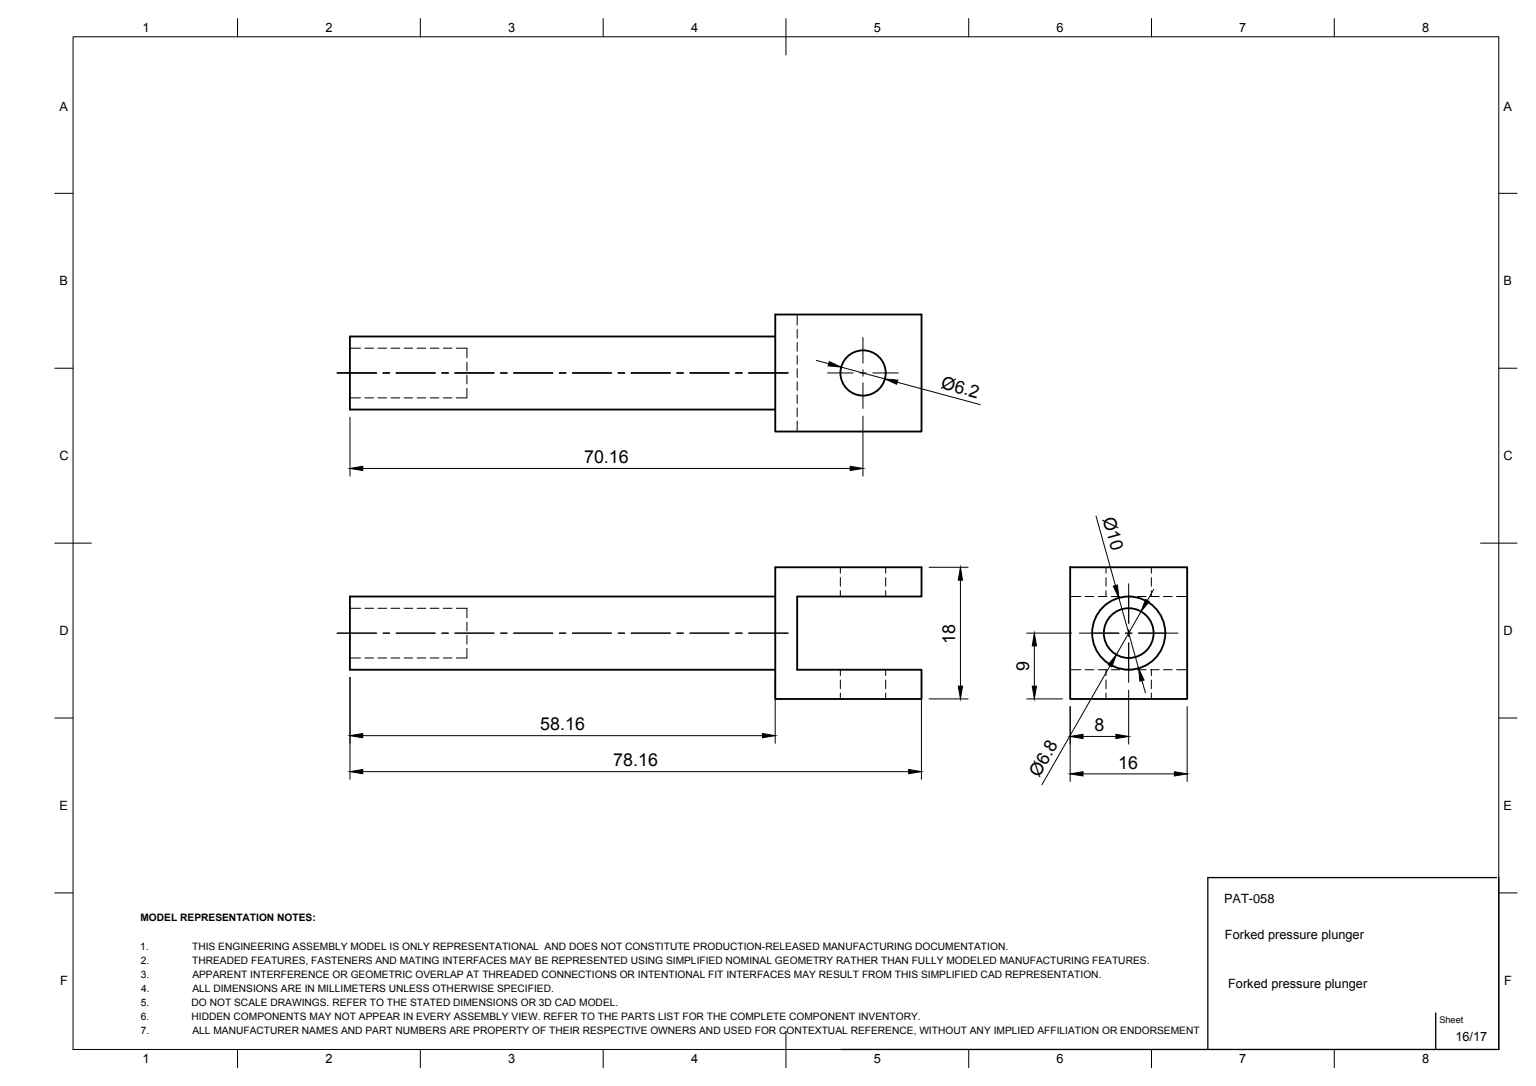
ISO-10303-21;
HEADER;
/* Generated by software containing ST-Developer
 * from STEP Tools, Inc. (www.steptools.com) 
 */

FILE_DESCRIPTION(
/* description */ ('Horizontal push-pull toggle clamp'),
/* implementation_level */ '2;1');

FILE_NAME(
/* name */ 'Forked pressure plunger.step',
/* time_stamp */ '2026-10-27T21:21:09-07:00',
/* author */ (''),
/* organization */ (''),
/* preprocessor_version */ 'ST-DEVELOPER v20.2',
/* originating_system */ 'Autodesk Translation Framework v15.17.0.0',
/* authorisation */ '');

FILE_SCHEMA (('AUTOMOTIVE_DESIGN { 1 0 10303 214 3 1 1 }'));
ENDSEC;

DATA;
#10=MECHANICAL_DESIGN_GEOMETRIC_PRESENTATION_REPRESENTATION('',(#190),#4791);
#164=SHAPE_REPRESENTATION_RELATIONSHIP('SRR','None',#4870,#177);
#177=ADVANCED_BREP_SHAPE_REPRESENTATION('',(#202),#4783);
#190=STYLED_ITEM('',(#5009),#202);
#202=MANIFOLD_SOLID_BREP('Body1',#2635);
#240=FACE_BOUND('',#637,.T.);
#241=FACE_BOUND('',#640,.T.);
#242=FACE_BOUND('',#643,.T.);
#243=FACE_BOUND('',#646,.T.);
#244=FACE_BOUND('',#649,.T.);
#245=FACE_BOUND('',#652,.T.);
#321=PLANE('',#2939);
#322=PLANE('',#2946);
#323=PLANE('',#2947);
#324=PLANE('',#2948);
#325=PLANE('',#2949);
#326=PLANE('',#2950);
#327=PLANE('',#2951);
#328=PLANE('',#2953);
#329=PLANE('',#2954);
#330=PLANE('',#2955);
#331=PLANE('',#2956);
#332=PLANE('',#2959);
#450=FACE_OUTER_BOUND('',#631,.T.);
#451=FACE_OUTER_BOUND('',#632,.T.);
#452=FACE_OUTER_BOUND('',#633,.T.);
#453=FACE_OUTER_BOUND('',#634,.T.);
#454=FACE_OUTER_BOUND('',#635,.T.);
#455=FACE_OUTER_BOUND('',#636,.T.);
#456=FACE_OUTER_BOUND('',#638,.T.);
#457=FACE_OUTER_BOUND('',#639,.T.);
#458=FACE_OUTER_BOUND('',#641,.T.);
#459=FACE_OUTER_BOUND('',#642,.T.);
#460=FACE_OUTER_BOUND('',#644,.T.);
#461=FACE_OUTER_BOUND('',#645,.T.);
#462=FACE_OUTER_BOUND('',#647,.T.);
#463=FACE_OUTER_BOUND('',#648,.T.);
#464=FACE_OUTER_BOUND('',#650,.T.);
#465=FACE_OUTER_BOUND('',#651,.T.);
#631=EDGE_LOOP('',(#2185,#2186,#2187,#2188));
#632=EDGE_LOOP('',(#2189));
#633=EDGE_LOOP('',(#2190,#2191,#2192,#2193));
#634=EDGE_LOOP('',(#2194,#2195,#2196,#2197));
#635=EDGE_LOOP('',(#2198,#2199,#2200,#2201));
#636=EDGE_LOOP('',(#2202,#2203,#2204,#2205));
#637=EDGE_LOOP('',(#2206));
#638=EDGE_LOOP('',(#2207,#2208,#2209,#2210,#2211,#2212,#2213,#2214));
#639=EDGE_LOOP('',(#2215,#2216,#2217,#2218));
#640=EDGE_LOOP('',(#2219));
#641=EDGE_LOOP('',(#2220,#2221,#2222,#2223));
#642=EDGE_LOOP('',(#2224,#2225,#2226,#2227));
#643=EDGE_LOOP('',(#2228));
#644=EDGE_LOOP('',(#2229,#2230,#2231,#2232,#2233,#2234,#2235,#2236));
#645=EDGE_LOOP('',(#2237,#2238,#2239,#2240));
#646=EDGE_LOOP('',(#2241));
#647=EDGE_LOOP('',(#2242,#2243,#2244,#2245));
#648=EDGE_LOOP('',(#2246,#2247,#2248,#2249));
#649=EDGE_LOOP('',(#2250));
#650=EDGE_LOOP('',(#2251,#2252,#2253,#2254));
#651=EDGE_LOOP('',(#2255));
#652=EDGE_LOOP('',(#2256));
#759=CIRCLE('',#2937,0.34);
#760=CIRCLE('',#2938,0.34);
#761=CIRCLE('',#2941,0.31);
#762=CIRCLE('',#2942,0.31);
#763=CIRCLE('',#2944,0.31);
#764=CIRCLE('',#2945,0.31);
#765=CIRCLE('',#2952,0.5);
#766=CIRCLE('',#2958,0.5);
#948=LINE('',#4294,#1168);
#949=LINE('',#4301,#1169);
#950=LINE('',#4307,#1170);
#951=LINE('',#4312,#1171);
#952=LINE('',#4314,#1172);
#953=LINE('',#4316,#1173);
#954=LINE('',#4317,#1174);
#955=LINE('',#4321,#1175);
#956=LINE('',#4323,#1176);
#957=LINE('',#4325,#1177);
#958=LINE('',#4326,#1178);
#959=LINE('',#4329,#1179);
#960=LINE('',#4330,#1180);
#961=LINE('',#4332,#1181);
#962=LINE('',#4334,#1182);
#963=LINE('',#4336,#1183);
#964=LINE('',#4337,#1184);
#965=LINE('',#4341,#1185);
#966=LINE('',#4342,#1186);
#967=LINE('',#4343,#1187);
#968=LINE('',#4346,#1188);
#969=LINE('',#4347,#1189);
#970=LINE('',#4349,#1190);
#971=LINE('',#4353,#1191);
#972=LINE('',#4355,#1192);
#973=LINE('',#4356,#1193);
#974=LINE('',#4359,#1194);
#975=LINE('',#4364,#1195);
#1168=VECTOR('',#3524,0.34);
#1169=VECTOR('',#3533,0.31);
#1170=VECTOR('',#3540,0.31);
#1171=VECTOR('',#3545,1.);
#1172=VECTOR('',#3546,1.);
#1173=VECTOR('',#3547,1.);
#1174=VECTOR('',#3548,1.);
#1175=VECTOR('',#3551,1.);
#1176=VECTOR('',#3552,1.);
#1177=VECTOR('',#3553,1.);
#1178=VECTOR('',#3554,1.);
#1179=VECTOR('',#3557,1.);
#1180=VECTOR('',#3558,1.);
#1181=VECTOR('',#3559,1.);
#1182=VECTOR('',#3560,1.);
#1183=VECTOR('',#3561,1.);
#1184=VECTOR('',#3562,1.);
#1185=VECTOR('',#3565,1.);
#1186=VECTOR('',#3566,1.);
#1187=VECTOR('',#3567,1.);
#1188=VECTOR('',#3570,1.);
#1189=VECTOR('',#3571,1.);
#1190=VECTOR('',#3574,1.);
#1191=VECTOR('',#3579,1.);
#1192=VECTOR('',#3580,1.);
#1193=VECTOR('',#3581,1.);
#1194=VECTOR('',#3586,1.);
#1195=VECTOR('',#3593,0.5);
#1369=VERTEX_POINT('',#4291);
#1370=VERTEX_POINT('',#4293);
#1371=VERTEX_POINT('',#4298);
#1372=VERTEX_POINT('',#4300);
#1373=VERTEX_POINT('',#4304);
#1374=VERTEX_POINT('',#4306);
#1375=VERTEX_POINT('',#4310);
#1376=VERTEX_POINT('',#4311);
#1377=VERTEX_POINT('',#4313);
#1378=VERTEX_POINT('',#4315);
#1379=VERTEX_POINT('',#4319);
#1380=VERTEX_POINT('',#4320);
#1381=VERTEX_POINT('',#4322);
#1382=VERTEX_POINT('',#4324);
#1383=VERTEX_POINT('',#4328);
#1384=VERTEX_POINT('',#4331);
#1385=VERTEX_POINT('',#4333);
#1386=VERTEX_POINT('',#4335);
#1387=VERTEX_POINT('',#4339);
#1388=VERTEX_POINT('',#4340);
#1389=VERTEX_POINT('',#4345);
#1390=VERTEX_POINT('',#4350);
#1391=VERTEX_POINT('',#4354);
#1392=VERTEX_POINT('',#4362);
#1654=EDGE_CURVE('',#1369,#1369,#759,.T.);
#1655=EDGE_CURVE('',#1369,#1370,#948,.T.);
#1656=EDGE_CURVE('',#1370,#1370,#760,.T.);
#1657=EDGE_CURVE('',#1371,#1371,#761,.T.);
#1658=EDGE_CURVE('',#1371,#1372,#949,.T.);
#1659=EDGE_CURVE('',#1372,#1372,#762,.T.);
#1660=EDGE_CURVE('',#1373,#1373,#763,.T.);
#1661=EDGE_CURVE('',#1373,#1374,#950,.T.);
#1662=EDGE_CURVE('',#1374,#1374,#764,.T.);
#1663=EDGE_CURVE('',#1375,#1376,#951,.T.);
#1664=EDGE_CURVE('',#1377,#1375,#952,.T.);
#1665=EDGE_CURVE('',#1378,#1377,#953,.T.);
#1666=EDGE_CURVE('',#1378,#1376,#954,.T.);
#1667=EDGE_CURVE('',#1379,#1380,#955,.T.);
#1668=EDGE_CURVE('',#1380,#1381,#956,.T.);
#1669=EDGE_CURVE('',#1381,#1382,#957,.T.);
#1670=EDGE_CURVE('',#1382,#1379,#958,.T.);
#1671=EDGE_CURVE('',#1383,#1375,#959,.T.);
#1672=EDGE_CURVE('',#1383,#1380,#960,.T.);
#1673=EDGE_CURVE('',#1384,#1379,#961,.T.);
#1674=EDGE_CURVE('',#1385,#1384,#962,.T.);
#1675=EDGE_CURVE('',#1385,#1386,#963,.T.);
#1676=EDGE_CURVE('',#1377,#1386,#964,.T.);
#1677=EDGE_CURVE('',#1387,#1388,#965,.T.);
#1678=EDGE_CURVE('',#1388,#1385,#966,.T.);
#1679=EDGE_CURVE('',#1384,#1387,#967,.T.);
#1680=EDGE_CURVE('',#1389,#1383,#968,.T.);
#1681=EDGE_CURVE('',#1389,#1381,#969,.T.);
#1682=EDGE_CURVE('',#1387,#1382,#970,.T.);
#1683=EDGE_CURVE('',#1390,#1390,#765,.T.);
#1684=EDGE_CURVE('',#1376,#1389,#971,.T.);
#1685=EDGE_CURVE('',#1391,#1378,#972,.T.);
#1686=EDGE_CURVE('',#1388,#1391,#973,.T.);
#1687=EDGE_CURVE('',#1386,#1391,#974,.T.);
#1688=EDGE_CURVE('',#1392,#1392,#766,.T.);
#1689=EDGE_CURVE('',#1392,#1390,#975,.T.);
#2185=ORIENTED_EDGE('',*,*,#1654,.F.);
#2186=ORIENTED_EDGE('',*,*,#1655,.T.);
#2187=ORIENTED_EDGE('',*,*,#1656,.F.);
#2188=ORIENTED_EDGE('',*,*,#1655,.F.);
#2189=ORIENTED_EDGE('',*,*,#1654,.T.);
#2190=ORIENTED_EDGE('',*,*,#1657,.F.);
#2191=ORIENTED_EDGE('',*,*,#1658,.T.);
#2192=ORIENTED_EDGE('',*,*,#1659,.F.);
#2193=ORIENTED_EDGE('',*,*,#1658,.F.);
#2194=ORIENTED_EDGE('',*,*,#1660,.F.);
#2195=ORIENTED_EDGE('',*,*,#1661,.T.);
#2196=ORIENTED_EDGE('',*,*,#1662,.F.);
#2197=ORIENTED_EDGE('',*,*,#1661,.F.);
#2198=ORIENTED_EDGE('',*,*,#1663,.F.);
#2199=ORIENTED_EDGE('',*,*,#1664,.F.);
#2200=ORIENTED_EDGE('',*,*,#1665,.F.);
#2201=ORIENTED_EDGE('',*,*,#1666,.T.);
#2202=ORIENTED_EDGE('',*,*,#1667,.T.);
#2203=ORIENTED_EDGE('',*,*,#1668,.T.);
#2204=ORIENTED_EDGE('',*,*,#1669,.T.);
#2205=ORIENTED_EDGE('',*,*,#1670,.T.);
#2206=ORIENTED_EDGE('',*,*,#1662,.T.);
#2207=ORIENTED_EDGE('',*,*,#1671,.F.);
#2208=ORIENTED_EDGE('',*,*,#1672,.T.);
#2209=ORIENTED_EDGE('',*,*,#1667,.F.);
#2210=ORIENTED_EDGE('',*,*,#1673,.F.);
#2211=ORIENTED_EDGE('',*,*,#1674,.F.);
#2212=ORIENTED_EDGE('',*,*,#1675,.T.);
#2213=ORIENTED_EDGE('',*,*,#1676,.F.);
#2214=ORIENTED_EDGE('',*,*,#1664,.T.);
#2215=ORIENTED_EDGE('',*,*,#1677,.T.);
#2216=ORIENTED_EDGE('',*,*,#1678,.T.);
#2217=ORIENTED_EDGE('',*,*,#1674,.T.);
#2218=ORIENTED_EDGE('',*,*,#1679,.T.);
#2219=ORIENTED_EDGE('',*,*,#1657,.T.);
#2220=ORIENTED_EDGE('',*,*,#1680,.F.);
#2221=ORIENTED_EDGE('',*,*,#1681,.T.);
#2222=ORIENTED_EDGE('',*,*,#1668,.F.);
#2223=ORIENTED_EDGE('',*,*,#1672,.F.);
#2224=ORIENTED_EDGE('',*,*,#1673,.T.);
#2225=ORIENTED_EDGE('',*,*,#1670,.F.);
#2226=ORIENTED_EDGE('',*,*,#1682,.F.);
#2227=ORIENTED_EDGE('',*,*,#1679,.F.);
#2228=ORIENTED_EDGE('',*,*,#1683,.F.);
#2229=ORIENTED_EDGE('',*,*,#1669,.F.);
#2230=ORIENTED_EDGE('',*,*,#1681,.F.);
#2231=ORIENTED_EDGE('',*,*,#1684,.F.);
#2232=ORIENTED_EDGE('',*,*,#1666,.F.);
#2233=ORIENTED_EDGE('',*,*,#1685,.F.);
#2234=ORIENTED_EDGE('',*,*,#1686,.F.);
#2235=ORIENTED_EDGE('',*,*,#1677,.F.);
#2236=ORIENTED_EDGE('',*,*,#1682,.T.);
#2237=ORIENTED_EDGE('',*,*,#1663,.T.);
#2238=ORIENTED_EDGE('',*,*,#1684,.T.);
#2239=ORIENTED_EDGE('',*,*,#1680,.T.);
#2240=ORIENTED_EDGE('',*,*,#1671,.T.);
#2241=ORIENTED_EDGE('',*,*,#1660,.T.);
#2242=ORIENTED_EDGE('',*,*,#1678,.F.);
#2243=ORIENTED_EDGE('',*,*,#1686,.T.);
#2244=ORIENTED_EDGE('',*,*,#1687,.F.);
#2245=ORIENTED_EDGE('',*,*,#1675,.F.);
#2246=ORIENTED_EDGE('',*,*,#1665,.T.);
#2247=ORIENTED_EDGE('',*,*,#1676,.T.);
#2248=ORIENTED_EDGE('',*,*,#1687,.T.);
#2249=ORIENTED_EDGE('',*,*,#1685,.T.);
#2250=ORIENTED_EDGE('',*,*,#1659,.T.);
#2251=ORIENTED_EDGE('',*,*,#1688,.F.);
#2252=ORIENTED_EDGE('',*,*,#1689,.T.);
#2253=ORIENTED_EDGE('',*,*,#1683,.T.);
#2254=ORIENTED_EDGE('',*,*,#1689,.F.);
#2255=ORIENTED_EDGE('',*,*,#1688,.T.);
#2256=ORIENTED_EDGE('',*,*,#1656,.T.);
#2463=CYLINDRICAL_SURFACE('',#2936,0.34);
#2464=CYLINDRICAL_SURFACE('',#2940,0.31);
#2465=CYLINDRICAL_SURFACE('',#2943,0.31);
#2466=CYLINDRICAL_SURFACE('',#2957,0.5);
#2566=ADVANCED_FACE('',(#450),#2463,.F.);
#2567=ADVANCED_FACE('',(#451),#321,.T.);
#2568=ADVANCED_FACE('',(#452),#2464,.F.);
#2569=ADVANCED_FACE('',(#453),#2465,.F.);
#2570=ADVANCED_FACE('',(#454),#322,.T.);
#2571=ADVANCED_FACE('',(#455,#240),#323,.T.);
#2572=ADVANCED_FACE('',(#456),#324,.T.);
#2573=ADVANCED_FACE('',(#457,#241),#325,.F.);
#2574=ADVANCED_FACE('',(#458),#326,.T.);
#2575=ADVANCED_FACE('',(#459,#242),#327,.T.);
#2576=ADVANCED_FACE('',(#460),#328,.T.);
#2577=ADVANCED_FACE('',(#461,#243),#329,.F.);
#2578=ADVANCED_FACE('',(#462),#330,.T.);
#2579=ADVANCED_FACE('',(#463,#244),#331,.T.);
#2580=ADVANCED_FACE('',(#464),#2466,.T.);
#2581=ADVANCED_FACE('',(#465,#245),#332,.T.);
#2635=CLOSED_SHELL('',(#2566,#2567,#2568,#2569,#2570,#2571,#2572,#2573,
#2574,#2575,#2576,#2577,#2578,#2579,#2580,#2581));
#2935=AXIS2_PLACEMENT_3D('',#4289,#3518,#3519);
#2936=AXIS2_PLACEMENT_3D('',#4290,#3520,#3521);
#2937=AXIS2_PLACEMENT_3D('',#4292,#3522,#3523);
#2938=AXIS2_PLACEMENT_3D('',#4295,#3525,#3526);
#2939=AXIS2_PLACEMENT_3D('',#4296,#3527,#3528);
#2940=AXIS2_PLACEMENT_3D('',#4297,#3529,#3530);
#2941=AXIS2_PLACEMENT_3D('',#4299,#3531,#3532);
#2942=AXIS2_PLACEMENT_3D('',#4302,#3534,#3535);
#2943=AXIS2_PLACEMENT_3D('',#4303,#3536,#3537);
#2944=AXIS2_PLACEMENT_3D('',#4305,#3538,#3539);
#2945=AXIS2_PLACEMENT_3D('',#4308,#3541,#3542);
#2946=AXIS2_PLACEMENT_3D('',#4309,#3543,#3544);
#2947=AXIS2_PLACEMENT_3D('',#4318,#3549,#3550);
#2948=AXIS2_PLACEMENT_3D('',#4327,#3555,#3556);
#2949=AXIS2_PLACEMENT_3D('',#4338,#3563,#3564);
#2950=AXIS2_PLACEMENT_3D('',#4344,#3568,#3569);
#2951=AXIS2_PLACEMENT_3D('',#4348,#3572,#3573);
#2952=AXIS2_PLACEMENT_3D('',#4351,#3575,#3576);
#2953=AXIS2_PLACEMENT_3D('',#4352,#3577,#3578);
#2954=AXIS2_PLACEMENT_3D('',#4357,#3582,#3583);
#2955=AXIS2_PLACEMENT_3D('',#4358,#3584,#3585);
#2956=AXIS2_PLACEMENT_3D('',#4360,#3587,#3588);
#2957=AXIS2_PLACEMENT_3D('',#4361,#3589,#3590);
#2958=AXIS2_PLACEMENT_3D('',#4363,#3591,#3592);
#2959=AXIS2_PLACEMENT_3D('',#4365,#3594,#3595);
#3518=DIRECTION('axis',(0.,0.,1.));
#3519=DIRECTION('refdir',(1.,0.,0.));
#3520=DIRECTION('center_axis',(1.,0.,0.));
#3521=DIRECTION('ref_axis',(0.,0.,-1.));
#3522=DIRECTION('center_axis',(1.,0.,0.));
#3523=DIRECTION('ref_axis',(0.,0.,-1.));
#3524=DIRECTION('',(1.,0.,0.));
#3525=DIRECTION('center_axis',(-1.,0.,0.));
#3526=DIRECTION('ref_axis',(0.,0.,-1.));
#3527=DIRECTION('center_axis',(1.,0.,0.));
#3528=DIRECTION('ref_axis',(0.,0.,-1.));
#3529=DIRECTION('center_axis',(0.,1.,0.));
#3530=DIRECTION('ref_axis',(1.,0.,0.));
#3531=DIRECTION('center_axis',(0.,1.,0.));
#3532=DIRECTION('ref_axis',(1.,0.,0.));
#3533=DIRECTION('',(0.,1.,0.));
#3534=DIRECTION('center_axis',(0.,-1.,0.));
#3535=DIRECTION('ref_axis',(1.,0.,0.));
#3536=DIRECTION('center_axis',(0.,1.,0.));
#3537=DIRECTION('ref_axis',(1.,0.,0.));
#3538=DIRECTION('center_axis',(0.,1.,0.));
#3539=DIRECTION('ref_axis',(1.,0.,0.));
#3540=DIRECTION('',(0.,1.,0.));
#3541=DIRECTION('center_axis',(0.,-1.,0.));
#3542=DIRECTION('ref_axis',(1.,0.,0.));
#3543=DIRECTION('center_axis',(-1.,0.,0.));
#3544=DIRECTION('ref_axis',(0.,0.,1.));
#3545=DIRECTION('',(0.,0.,1.));
#3546=DIRECTION('',(0.,1.,0.));
#3547=DIRECTION('',(0.,0.,-1.));
#3548=DIRECTION('',(0.,1.,0.));
#3549=DIRECTION('center_axis',(0.,1.,0.));
#3550=DIRECTION('ref_axis',(0.,0.,1.));
#3551=DIRECTION('',(-1.,0.,0.));
#3552=DIRECTION('',(0.,0.,1.));
#3553=DIRECTION('',(1.,0.,0.));
#3554=DIRECTION('',(0.,0.,-1.));
#3555=DIRECTION('center_axis',(0.,0.,-1.));
#3556=DIRECTION('ref_axis',(-1.,0.,0.));
#3557=DIRECTION('',(1.,0.,0.));
#3558=DIRECTION('',(0.,1.,0.));
#3559=DIRECTION('',(0.,1.,0.));
#3560=DIRECTION('',(1.,0.,0.));
#3561=DIRECTION('',(0.,1.,0.));
#3562=DIRECTION('',(-1.,0.,0.));
#3563=DIRECTION('center_axis',(0.,1.,0.));
#3564=DIRECTION('ref_axis',(1.,0.,0.));
#3565=DIRECTION('',(-1.,0.,0.));
#3566=DIRECTION('',(0.,0.,-1.));
#3567=DIRECTION('',(0.,0.,1.));
#3568=DIRECTION('center_axis',(-1.,0.,0.));
#3569=DIRECTION('ref_axis',(0.,0.,1.));
#3570=DIRECTION('',(0.,0.,-1.));
#3571=DIRECTION('',(0.,1.,0.));
#3572=DIRECTION('center_axis',(1.,0.,0.));
#3573=DIRECTION('ref_axis',(0.,0.,-1.));
#3574=DIRECTION('',(0.,1.,0.));
#3575=DIRECTION('center_axis',(1.,0.,0.));
#3576=DIRECTION('ref_axis',(0.,0.,-1.));
#3577=DIRECTION('center_axis',(0.,0.,1.));
#3578=DIRECTION('ref_axis',(1.,0.,0.));
#3579=DIRECTION('',(-1.,0.,0.));
#3580=DIRECTION('',(1.,0.,0.));
#3581=DIRECTION('',(0.,1.,0.));
#3582=DIRECTION('center_axis',(0.,1.,0.));
#3583=DIRECTION('ref_axis',(1.,0.,0.));
#3584=DIRECTION('center_axis',(-1.,0.,0.));
#3585=DIRECTION('ref_axis',(0.,0.,1.));
#3586=DIRECTION('',(0.,0.,1.));
#3587=DIRECTION('center_axis',(0.,1.,0.));
#3588=DIRECTION('ref_axis',(0.,0.,1.));
#3589=DIRECTION('center_axis',(1.,0.,0.));
#3590=DIRECTION('ref_axis',(0.,0.,-1.));
#3591=DIRECTION('center_axis',(1.,0.,0.));
#3592=DIRECTION('ref_axis',(0.,0.,-1.));
#3593=DIRECTION('',(-1.,0.,0.));
#3594=DIRECTION('center_axis',(1.,0.,0.));
#3595=DIRECTION('ref_axis',(0.,0.,-1.));
#4289=CARTESIAN_POINT('',(0.,0.,0.));
#4290=CARTESIAN_POINT('Origin',(11.4,0.,2.5));
#4291=CARTESIAN_POINT('',(11.4,-4.163799117101E-17,2.84));
#4292=CARTESIAN_POINT('Origin',(11.4,0.,2.5));
#4293=CARTESIAN_POINT('',(13.,4.163799117101E-17,2.84));
#4294=CARTESIAN_POINT('',(11.4,-4.163799117101E-17,2.84));
#4295=CARTESIAN_POINT('Origin',(13.,0.,2.5));
#4296=CARTESIAN_POINT('Origin',(11.4,0.,2.5));
#4297=CARTESIAN_POINT('Origin',(5.98369790806552,-1.,2.5));
#4298=CARTESIAN_POINT('',(5.67369790806552,-0.9,2.5));
#4299=CARTESIAN_POINT('Origin',(5.98369790806552,-0.9,2.5));
#4300=CARTESIAN_POINT('',(5.67369790806552,-0.5,2.5));
#4301=CARTESIAN_POINT('',(5.67369790806552,-1.,2.5));
#4302=CARTESIAN_POINT('Origin',(5.98369790806552,-0.5,2.5));
#4303=CARTESIAN_POINT('Origin',(5.98369790806552,-1.,2.5));
#4304=CARTESIAN_POINT('',(5.67369790806552,0.5,2.5));
#4305=CARTESIAN_POINT('Origin',(5.98369790806552,0.5,2.5));
#4306=CARTESIAN_POINT('',(5.67369790806552,0.9,2.5));
#4307=CARTESIAN_POINT('',(5.67369790806552,-1.,2.5));
#4308=CARTESIAN_POINT('Origin',(5.98369790806552,0.9,2.5));
#4309=CARTESIAN_POINT('Origin',(6.88369790806552,-0.9,1.7));
#4310=CARTESIAN_POINT('',(6.88369790806552,0.5,1.7));
#4311=CARTESIAN_POINT('',(6.88369790806552,0.5,3.3));
#4312=CARTESIAN_POINT('',(6.88369790806552,0.5,2.1));
#4313=CARTESIAN_POINT('',(6.88369790806552,-0.5,1.7));
#4314=CARTESIAN_POINT('',(6.88369790806552,-0.9,1.7));
#4315=CARTESIAN_POINT('',(6.88369790806552,-0.5,3.3));
#4316=CARTESIAN_POINT('',(6.88369790806552,-0.5,2.1));
#4317=CARTESIAN_POINT('',(6.88369790806552,-0.9,3.3));
#4318=CARTESIAN_POINT('Origin',(6.18369790806552,0.9,2.5));
#4319=CARTESIAN_POINT('',(7.18369790806552,0.9,1.7));
#4320=CARTESIAN_POINT('',(5.18369790806552,0.9,1.7));
#4321=CARTESIAN_POINT('',(5.18369790806552,0.9,1.7));
#4322=CARTESIAN_POINT('',(5.18369790806552,0.9,3.3));
#4323=CARTESIAN_POINT('',(5.18369790806552,0.9,3.3));
#4324=CARTESIAN_POINT('',(7.18369790806552,0.9,3.3));
#4325=CARTESIAN_POINT('',(7.18369790806552,0.9,3.3));
#4326=CARTESIAN_POINT('',(7.18369790806552,0.9,1.7));
#4327=CARTESIAN_POINT('Origin',(7.18369790806552,0.5,1.7));
#4328=CARTESIAN_POINT('',(5.18369790806552,0.5,1.7));
#4329=CARTESIAN_POINT('',(5.18369790806552,0.5,1.7));
#4330=CARTESIAN_POINT('',(5.18369790806552,0.5,1.7));
#4331=CARTESIAN_POINT('',(7.18369790806552,-0.9,1.7));
#4332=CARTESIAN_POINT('',(7.18369790806552,0.5,1.7));
#4333=CARTESIAN_POINT('',(5.18369790806552,-0.9,1.7));
#4334=CARTESIAN_POINT('',(5.18369790806552,-0.9,1.7));
#4335=CARTESIAN_POINT('',(5.18369790806552,-0.5,1.7));
#4336=CARTESIAN_POINT('',(5.18369790806552,-0.9,1.7));
#4337=CARTESIAN_POINT('',(5.18369790806552,-0.5,1.7));
#4338=CARTESIAN_POINT('Origin',(6.18369790806552,-0.9,2.5));
#4339=CARTESIAN_POINT('',(7.18369790806552,-0.9,3.3));
#4340=CARTESIAN_POINT('',(5.18369790806552,-0.9,3.3));
#4341=CARTESIAN_POINT('',(7.18369790806552,-0.9,3.3));
#4342=CARTESIAN_POINT('',(5.18369790806552,-0.9,3.3));
#4343=CARTESIAN_POINT('',(7.18369790806552,-0.9,1.7));
#4344=CARTESIAN_POINT('Origin',(5.18369790806552,0.5,1.7));
#4345=CARTESIAN_POINT('',(5.18369790806552,0.5,3.3));
#4346=CARTESIAN_POINT('',(5.18369790806552,0.5,3.3));
#4347=CARTESIAN_POINT('',(5.18369790806552,0.5,3.3));
#4348=CARTESIAN_POINT('Origin',(7.18369790806552,0.5,3.3));
#4349=CARTESIAN_POINT('',(7.18369790806552,0.5,3.3));
#4350=CARTESIAN_POINT('',(7.18369790806552,-6.12323399573677E-17,3.));
#4351=CARTESIAN_POINT('Origin',(7.18369790806552,0.,2.5));
#4352=CARTESIAN_POINT('Origin',(5.18369790806552,0.5,3.3));
#4353=CARTESIAN_POINT('',(7.18369790806552,0.5,3.3));
#4354=CARTESIAN_POINT('',(5.18369790806552,-0.5,3.3));
#4355=CARTESIAN_POINT('',(7.18369790806552,-0.5,3.3));
#4356=CARTESIAN_POINT('',(5.18369790806552,-0.9,3.3));
#4357=CARTESIAN_POINT('Origin',(6.18369790806552,0.5,2.5));
#4358=CARTESIAN_POINT('Origin',(5.18369790806552,-0.9,1.7));
#4359=CARTESIAN_POINT('',(5.18369790806552,-0.5,3.3));
#4360=CARTESIAN_POINT('Origin',(6.18369790806552,-0.5,2.5));
#4361=CARTESIAN_POINT('Origin',(6.98369791,0.,2.5));
#4362=CARTESIAN_POINT('',(13.,-6.12323399573677E-17,3.));
#4363=CARTESIAN_POINT('Origin',(13.,0.,2.5));
#4364=CARTESIAN_POINT('',(6.98369791,-6.12323399573677E-17,3.));
#4365=CARTESIAN_POINT('Origin',(13.,0.,2.5));
#4764=UNCERTAINTY_MEASURE_WITH_UNIT(LENGTH_MEASURE(0.001),#4792,
'DISTANCE_ACCURACY_VALUE',
'Maximum model space distance between geometric entities at asserted c
onnectivities');
#4772=UNCERTAINTY_MEASURE_WITH_UNIT(LENGTH_MEASURE(0.001),#4792,
'DISTANCE_ACCURACY_VALUE',
'Maximum model space distance between geometric entities at asserted c
onnectivities');
#4783=(
GEOMETRIC_REPRESENTATION_CONTEXT(3)
GLOBAL_UNCERTAINTY_ASSIGNED_CONTEXT((#4764))
GLOBAL_UNIT_ASSIGNED_CONTEXT((#4792,#4794,#4795))
REPRESENTATION_CONTEXT('','3D')
);
#4791=(
GEOMETRIC_REPRESENTATION_CONTEXT(3)
GLOBAL_UNCERTAINTY_ASSIGNED_CONTEXT((#4772))
GLOBAL_UNIT_ASSIGNED_CONTEXT((#4792,#4794,#4795))
REPRESENTATION_CONTEXT('','3D')
);
#4792=(
LENGTH_UNIT()
NAMED_UNIT(*)
SI_UNIT(.CENTI.,.METRE.)
);
#4794=(
NAMED_UNIT(*)
PLANE_ANGLE_UNIT()
SI_UNIT($,.RADIAN.)
);
#4795=(
NAMED_UNIT(*)
SI_UNIT($,.STERADIAN.)
SOLID_ANGLE_UNIT()
);
#4806=SHAPE_DEFINITION_REPRESENTATION(#4825,#4870);
#4825=PRODUCT_DEFINITION_SHAPE('',$,#4889);
#4870=SHAPE_REPRESENTATION('',(#2935),#4783);
#4878=PRODUCT_DEFINITION_CONTEXT('part definition',#4934,'design');
#4889=PRODUCT_DEFINITION('Forked pressure plunger',
'Forked pressure plunger',#4907,#4878);
#4907=PRODUCT_DEFINITION_FORMATION('',$,#4946);
#4934=APPLICATION_CONTEXT(
'Core Data for Automotive Mechanical Design Process');
#4935=PRODUCT_CONTEXT('part definition',#4934,'mechanical');
#4946=PRODUCT('Forked pressure plunger','Forked pressure plunger',
'Forked pressure plunger',(#4935));
#5003=COLOUR_RGB('Light Blue',0.38,0.62,0.78);
#5004=FILL_AREA_STYLE_COLOUR('',#5003);
#5005=FILL_AREA_STYLE('',(#5004));
#5006=SURFACE_STYLE_FILL_AREA(#5005);
#5007=SURFACE_SIDE_STYLE('',(#5006));
#5008=SURFACE_STYLE_USAGE(.BOTH.,#5007);
#5009=PRESENTATION_STYLE_ASSIGNMENT((#5008));
ENDSEC;
END-ISO-10303-21;
